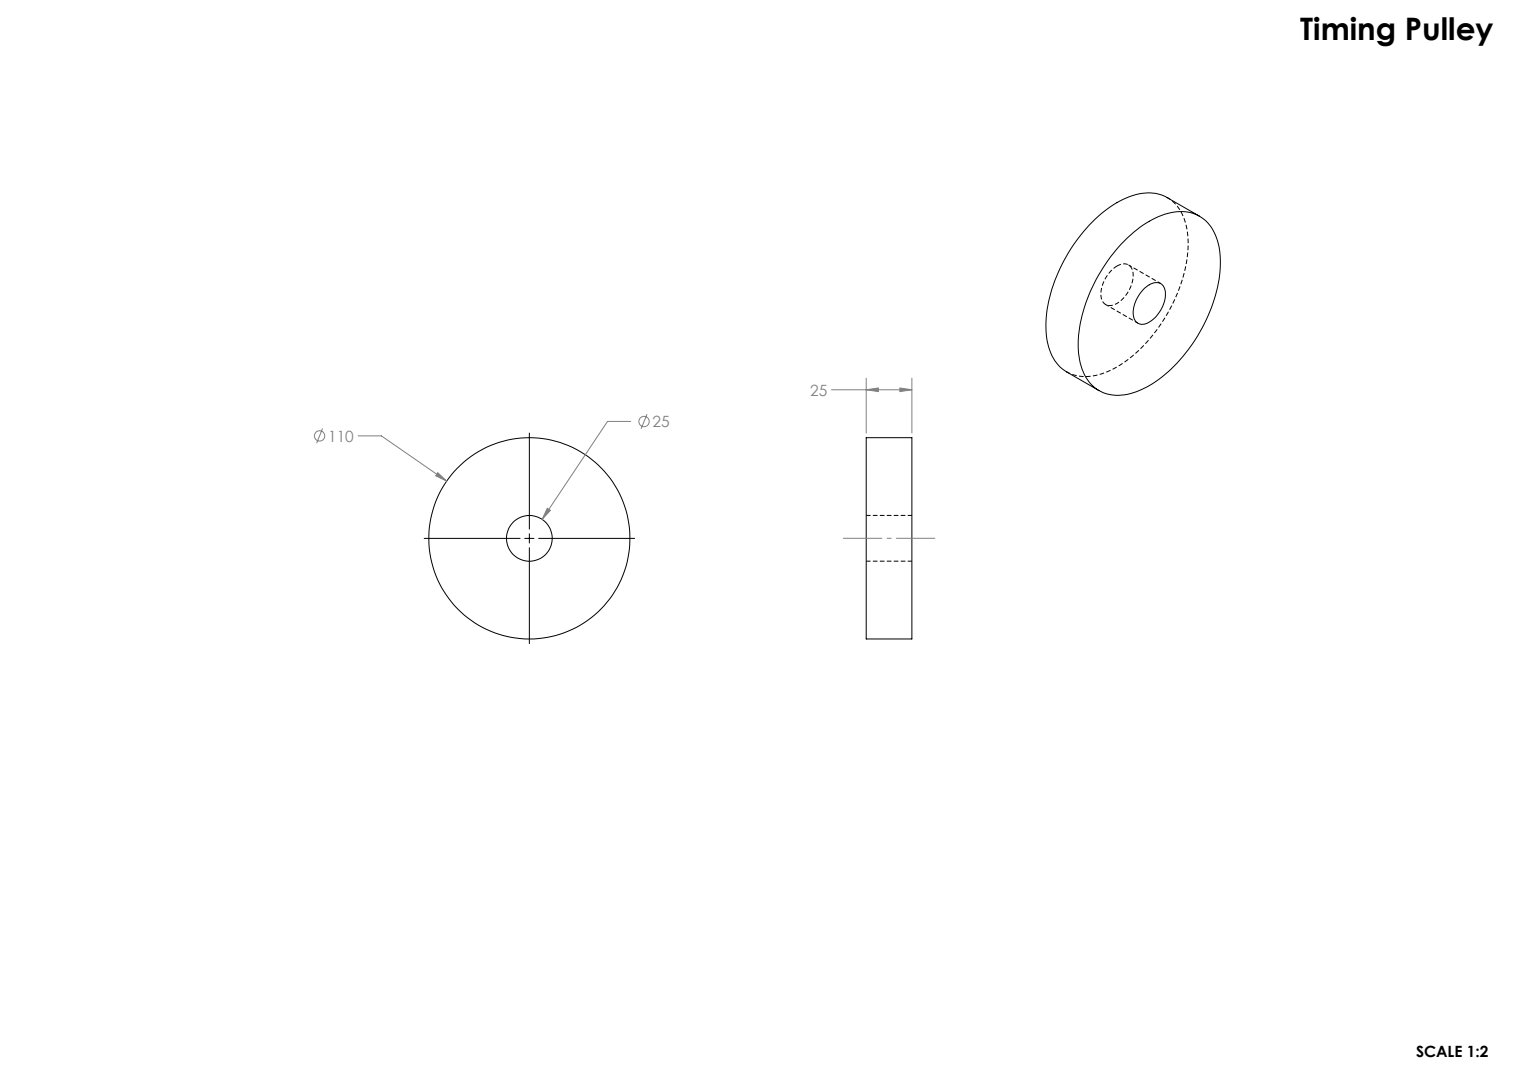
ISO-10303-21;
HEADER;
FILE_DESCRIPTION (('STEP AP214'),
    '1' );
FILE_NAME ('Timing Pulley.step',
    '2026-10-28T15:55:38',
    ( '' ),
    ( '' ),
    'SwSTEP 2.0',
    'SolidWorks 2025',
    '' );
FILE_SCHEMA (( 'AUTOMOTIVE_DESIGN' ));
ENDSEC;

DATA;
#97=ADVANCED_FACE ( 'NONE', ( #330, #202 ), #6713, .F. ) ;
#161=CARTESIAN_POINT ( 'NONE',  ( 5.551115123125782702E-14, 12.49999999999999645, -1.387778780781445676E-14 ) ) ;
#202=FACE_OUTER_BOUND ( 'NONE', #7839, .T. ) ;
#330=FACE_BOUND ( 'NONE', #1932, .T. ) ;
#354=VERTEX_POINT ( 'NONE', #1827 ) ;
#402=VERTEX_POINT ( 'NONE', #4592 ) ;
#516=AXIS2_PLACEMENT_3D ( 'NONE', #7483, #1692, #2897 ) ;
#543=CARTESIAN_POINT ( 'NONE',  ( 5.551115123125782702E-14, 12.49999999999999645, -1.387778780781445676E-14 ) ) ;
#563=AXIS2_PLACEMENT_3D ( 'NONE', #1559, #5435, #1598 ) ;
#639=AXIS2_PLACEMENT_3D ( 'NONE', #5635, #1167, #8220 ) ;
#714=DIRECTION ( 'NONE',  ( -1.752490724247359037E-17, 1.000000000000000000, 3.853078496550133260E-17 ) ) ;
#722=CARTESIAN_POINT ( 'NONE',  ( 5.551115123125782702E-14, 12.50000000000001066, -1.387778780781445676E-14 ) ) ;
#835=CARTESIAN_POINT ( 'NONE',  ( -1.173433385984103696E-13, -12.50000000000001066, -12.49999999999998757 ) ) ;
#854=VECTOR ( 'NONE', #4682, 1000.000000000000000 ) ;
#961=DIRECTION ( 'NONE',  ( 6.106226635438364917E-16, 3.154042683594196846E-17, 1.000000000000000000 ) ) ;
#969=PRODUCT_DEFINITION ( 'UNKNOWN', '', #7047, #8011 ) ;
#1020=ORIENTED_EDGE ( 'NONE', *, *, #2382, .F. ) ;
#1091=PRODUCT ( 'Timing Pulley', 'Timing Pulley', '', ( #7475 ) ) ;
#1167=DIRECTION ( 'NONE',  ( -1.752490724247359037E-17, 1.000000000000000000, 3.853078496550133260E-17 ) ) ;
#1272=CARTESIAN_POINT ( 'NONE',  ( -1.033895191682177028E-13, -12.50000000000001066, 12.50000000000000533 ) ) ;
#1299=AXIS2_PLACEMENT_3D ( 'NONE', #5884, #1507, #5927 ) ;
#1302=FACE_OUTER_BOUND ( 'NONE', #2125, .T. ) ;
#1306=CARTESIAN_POINT ( 'NONE',  ( -1.380900529026473240E-13, 12.49999999999999822, -55.00000000000001421 ) ) ;
#1313=ORIENTED_EDGE ( 'NONE', *, *, #1691, .T. ) ;
#1380=( LENGTH_UNIT ( ) NAMED_UNIT ( * ) SI_UNIT ( .MILLI., .METRE. ) );
#1422=ORIENTED_EDGE ( 'NONE', *, *, #7530, .F. ) ;
#1442=DIRECTION ( 'NONE',  ( 6.106226635438361958E-16, 0.000000000000000000, 1.000000000000000000 ) ) ;
#1481=( GEOMETRIC_REPRESENTATION_CONTEXT ( 3 ) GLOBAL_UNCERTAINTY_ASSIGNED_CONTEXT ( ( #5648 ) ) GLOBAL_UNIT_ASSIGNED_CONTEXT ( ( #2505, #4543, #3802 ) ) REPRESENTATION_CONTEXT ( 'NONE', 'WORKASPACE' ) );
#1501=ORIENTED_EDGE ( 'NONE', *, *, #6382, .F. ) ;
#1507=DIRECTION ( 'NONE',  ( 0.000000000000000000, 0.000000000000000000, 1.000000000000000000 ) ) ;
#1530=AXIS2_PLACEMENT_3D ( 'NONE', #2669, #2062, #2013 ) ;
#1559=CARTESIAN_POINT ( 'NONE',  ( -1.110223024625156540E-13, -12.49999999999999645, 1.387778780781445676E-14 ) ) ;
#1592=FACE_OUTER_BOUND ( 'NONE', #3238, .T. ) ;
#1598=DIRECTION ( 'NONE',  ( -6.106226635438364917E-16, -3.853078496550153598E-17, -1.000000000000000000 ) ) ;
#1650=DIRECTION ( 'NONE',  ( 6.106226635438361958E-16, 0.000000000000000000, 1.000000000000000000 ) ) ;
#1691=EDGE_CURVE ( 'NONE', #5627, #402, #6915, .T. ) ;
#1692=DIRECTION ( 'NONE',  ( -1.752490724247359037E-17, 1.000000000000000000, 3.853078496550133260E-17 ) ) ;
#1704=AXIS2_PLACEMENT_3D ( 'NONE', #2605, #5723, #8304 ) ;
#1705=DIRECTION ( 'NONE',  ( -1.752490724247359037E-17, 1.000000000000000000, 3.853078496550133260E-17 ) ) ;
#1733=VECTOR ( 'NONE', #5059, 1000.000000000000000 ) ;
#1752=ADVANCED_FACE ( 'NONE', ( #7099 ), #3846, .F. ) ;
#1780=EDGE_CURVE ( 'NONE', #5976, #2287, #7789, .T. ) ;
#1803=EDGE_CURVE ( 'NONE', #2287, #6267, #4623, .T. ) ;
#1827=CARTESIAN_POINT ( 'NONE',  ( -7.743805596760466869E-14, -12.49999999999999467, 54.99999999999997868 ) ) ;
#1884=CIRCLE ( 'NONE', #2423, 12.49999999999999289 ) ;
#1917=CARTESIAN_POINT ( 'NONE',  ( -7.743805596760466869E-14, -12.50000000000000888, 54.99999999999997868 ) ) ;
#1932=EDGE_LOOP ( 'NONE', ( #5556, #4034 ) ) ;
#1968=EDGE_CURVE ( 'NONE', #6651, #8339, #1884, .T. ) ;
#2013=DIRECTION ( 'NONE',  ( 6.106226635438364917E-16, 3.154042683594196846E-17, 1.000000000000000000 ) ) ;
#2062=DIRECTION ( 'NONE',  ( -1.752490724247359037E-17, 1.000000000000000000, 3.853078496550133260E-17 ) ) ;
#2125=EDGE_LOOP ( 'NONE', ( #7392, #3168, #5494, #5366 ) ) ;
#2287=VERTEX_POINT ( 'NONE', #1306 ) ;
#2300=CARTESIAN_POINT ( 'NONE',  ( 8.909539772616881237E-14, 12.49999999999999822, 54.99999999999995026 ) ) ;
#2382=EDGE_CURVE ( 'NONE', #402, #5627, #4177, .T. ) ;
#2398=ADVANCED_FACE ( 'NONE', ( #5522, #3511 ), #8130, .T. ) ;
#2423=AXIS2_PLACEMENT_3D ( 'NONE', #5830, #5321, #1442 ) ;
#2481=APPLICATION_CONTEXT ( 'automotive_design' ) ;
#2505=( LENGTH_UNIT ( ) NAMED_UNIT ( * ) SI_UNIT ( .MILLI., .METRE. ) );
#2512=CARTESIAN_POINT ( 'NONE',  ( -1.110223024625156540E-13, -12.50000000000001066, 1.387778780781445676E-14 ) ) ;
#2605=CARTESIAN_POINT ( 'NONE',  ( -1.110223024625156540E-13, -12.50000000000001066, 1.387778780781445676E-14 ) ) ;
#2607=AXIS2_PLACEMENT_3D ( 'NONE', #2512, #5752, #7022 ) ;
#2669=CARTESIAN_POINT ( 'NONE',  ( 5.551115123125782702E-14, 12.49999999999999645, -1.387778780781445676E-14 ) ) ;
#2741=DIRECTION ( 'NONE',  ( 1.752490724247363967E-17, -1.000000000000000000, 3.853078496550152365E-17 ) ) ;
#2796=AXIS2_PLACEMENT_3D ( 'NONE', #4981, #714, #5818 ) ;
#2897=DIRECTION ( 'NONE',  ( 6.106226635438364917E-16, 3.154042683594196846E-17, 1.000000000000000000 ) ) ;
#2966=CARTESIAN_POINT ( 'NONE',  ( -1.110223024625156540E-13, -12.50000000000001066, 1.387778780781445676E-14 ) ) ;
#3035=ADVANCED_FACE ( 'NONE', ( #1302 ), #6484, .T. ) ;
#3112=DIRECTION ( 'NONE',  ( -1.752490724247359037E-17, 1.000000000000000000, 3.853078496550133260E-17 ) ) ;
#3121=DIRECTION ( 'NONE',  ( -1.752490724247359037E-17, 1.000000000000000000, 3.853078496550133260E-17 ) ) ;
#3140=CYLINDRICAL_SURFACE ( 'NONE', #1704, 12.49999999999999289 ) ;
#3168=ORIENTED_EDGE ( 'NONE', *, *, #1780, .T. ) ;
#3185=UNCERTAINTY_MEASURE_WITH_UNIT (LENGTH_MEASURE( 1.000000000000000082E-05 ), #1380, 'distance_accuracy_value', 'NONE');
#3238=EDGE_LOOP ( 'NONE', ( #3403, #5267, #6886, #7093 ) ) ;
#3273=ORIENTED_EDGE ( 'NONE', *, *, #2382, .T. ) ;
#3372=ADVANCED_FACE ( 'NONE', ( #6988 ), #3140, .F. ) ;
#3403=ORIENTED_EDGE ( 'NONE', *, *, #1780, .F. ) ;
#3486=MECHANICAL_DESIGN_GEOMETRIC_PRESENTATION_REPRESENTATION('',(#7953),#1481);
#3511=FACE_OUTER_BOUND ( 'NONE', #5551, .T. ) ;
#3621=EDGE_LOOP ( 'NONE', ( #3273, #1313 ) ) ;
#3632=( NAMED_UNIT ( * ) PLANE_ANGLE_UNIT ( ) SI_UNIT ( $, .RADIAN. ) );
#3648=AXIS2_PLACEMENT_3D ( 'NONE', #3919, #6487, #4834 ) ;
#3708=PRODUCT_DEFINITION_SHAPE ( 'NONE', 'NONE',  #969 ) ;
#3729=CIRCLE ( 'NONE', #5885, 12.49999999999999289 ) ;
#3802=( NAMED_UNIT ( * ) SI_UNIT ( $, .STERADIAN. ) SOLID_ANGLE_UNIT ( ) );
#3846=CYLINDRICAL_SURFACE ( 'NONE', #2607, 12.49999999999999289 ) ;
#3890=CARTESIAN_POINT ( 'NONE',  ( -1.380900529026471473E-13, -12.49999999999999467, -54.99999999999998579 ) ) ;
#3905=CARTESIAN_POINT ( 'NONE',  ( -1.173433385984108997E-13, 12.50000000000001066, -12.50000000000001421 ) ) ;
#3919=CARTESIAN_POINT ( 'NONE',  ( -1.110223024625156540E-13, -12.50000000000001066, 1.387778780781445676E-14 ) ) ;
#3930=EDGE_CURVE ( 'NONE', #8339, #6651, #3729, .T. ) ;
#3965=SHAPE_REPRESENTATION ( 'Timing Pulley', ( #1299 ), #6550 ) ;
#3985=DIRECTION ( 'NONE',  ( -1.752490724247359037E-17, 1.000000000000000000, 3.853078496550133260E-17 ) ) ;
#4034=ORIENTED_EDGE ( 'NONE', *, *, #3930, .F. ) ;
#4091=EDGE_CURVE ( 'NONE', #354, #5976, #7375, .T. ) ;
#4132=CIRCLE ( 'NONE', #516, 54.99999999999996447 ) ;
#4177=CIRCLE ( 'NONE', #3648, 12.49999999999999289 ) ;
#4463=DIRECTION ( 'NONE',  ( 6.106226635438361958E-16, 0.000000000000000000, 1.000000000000000000 ) ) ;
#4480=CLOSED_SHELL ( 'NONE', ( #3035, #1752, #2398, #3372, #97, #5773 ) ) ;
#4541=LINE ( 'NONE', #1917, #1733 ) ;
#4543=( NAMED_UNIT ( * ) PLANE_ANGLE_UNIT ( ) SI_UNIT ( $, .RADIAN. ) );
#4581=ORIENTED_EDGE ( 'NONE', *, *, #4956, .F. ) ;
#4592=CARTESIAN_POINT ( 'NONE',  ( -1.033895191682177028E-13, -12.50000000000001066, 12.50000000000000533 ) ) ;
#4623=CIRCLE ( 'NONE', #1530, 54.99999999999996447 ) ;
#4666=ORIENTED_EDGE ( 'NONE', *, *, #6382, .T. ) ;
#4682=DIRECTION ( 'NONE',  ( -1.752490724247359037E-17, 1.000000000000000000, 3.853078496550133260E-17 ) ) ;
#4708=VECTOR ( 'NONE', #1705, 1000.000000000000000 ) ;
#4721=CARTESIAN_POINT ( 'NONE',  ( -1.110223024625156540E-13, -12.50000000000001066, 1.387778780781445676E-14 ) ) ;
#4764=DIRECTION ( 'NONE',  ( -6.106226635438364917E-16, -3.853078496550153598E-17, -1.000000000000000000 ) ) ;
#4834=DIRECTION ( 'NONE',  ( 6.106226635438361958E-16, 0.000000000000000000, 1.000000000000000000 ) ) ;
#4863=( NAMED_UNIT ( * ) SI_UNIT ( $, .STERADIAN. ) SOLID_ANGLE_UNIT ( ) );
#4956=EDGE_CURVE ( 'NONE', #5976, #354, #4132, .T. ) ;
#4966=AXIS2_PLACEMENT_3D ( 'NONE', #2966, #8003, #961 ) ;
#4981=CARTESIAN_POINT ( 'NONE',  ( -1.110223024625156540E-13, -12.50000000000001066, 1.387778780781445676E-14 ) ) ;
#5022=AXIS2_PLACEMENT_3D ( 'NONE', #4721, #6670, #1650 ) ;
#5059=DIRECTION ( 'NONE',  ( -1.752490724247359037E-17, 1.000000000000000000, 3.853078496550133260E-17 ) ) ;
#5061=ORIENTED_EDGE ( 'NONE', *, *, #7530, .T. ) ;
#5100=EDGE_CURVE ( 'NONE', #354, #6267, #4541, .T. ) ;
#5267=ORIENTED_EDGE ( 'NONE', *, *, #4956, .T. ) ;
#5321=DIRECTION ( 'NONE',  ( -1.752490724247359037E-17, 1.000000000000000000, 3.853078496550133260E-17 ) ) ;
#5366=ORIENTED_EDGE ( 'NONE', *, *, #5100, .F. ) ;
#5435=DIRECTION ( 'NONE',  ( 1.752490724247363967E-17, -1.000000000000000000, 3.853078496550152365E-17 ) ) ;
#5494=ORIENTED_EDGE ( 'NONE', *, *, #5515, .F. ) ;
#5505=LINE ( 'NONE', #6079, #4708 ) ;
#5515=EDGE_CURVE ( 'NONE', #6267, #2287, #8218, .T. ) ;
#5522=FACE_BOUND ( 'NONE', #3621, .T. ) ;
#5551=EDGE_LOOP ( 'NONE', ( #6960, #4581 ) ) ;
#5554=CYLINDRICAL_SURFACE ( 'NONE', #4966, 54.99999999999996447 ) ;
#5556=ORIENTED_EDGE ( 'NONE', *, *, #1968, .F. ) ;
#5627=VERTEX_POINT ( 'NONE', #835 ) ;
#5635=CARTESIAN_POINT ( 'NONE',  ( -1.110223024625156540E-13, -12.49999999999999645, 1.387778780781445676E-14 ) ) ;
#5648=UNCERTAINTY_MEASURE_WITH_UNIT (LENGTH_MEASURE( 1.000000000000000082E-05 ), #2505, 'distance_accuracy_value', 'NONE');
#5702=LINE ( 'NONE', #1272, #6053 ) ;
#5723=DIRECTION ( 'NONE',  ( -1.752490724247359037E-17, 1.000000000000000000, 3.853078496550133260E-17 ) ) ;
#5752=DIRECTION ( 'NONE',  ( -1.752490724247359037E-17, 1.000000000000000000, 3.853078496550133260E-17 ) ) ;
#5773=ADVANCED_FACE ( 'NONE', ( #1592 ), #5554, .T. ) ;
#5818=DIRECTION ( 'NONE',  ( 6.106226635438364917E-16, 3.154042683594196846E-17, 1.000000000000000000 ) ) ;
#5830=CARTESIAN_POINT ( 'NONE',  ( 5.551115123125782702E-14, 12.50000000000001066, -1.387778780781445676E-14 ) ) ;
#5860=APPLICATION_CONTEXT ( 'automotive_design' ) ;
#5884=CARTESIAN_POINT ( 'NONE',  ( 0.000000000000000000, 0.000000000000000000, 0.000000000000000000 ) ) ;
#5885=AXIS2_PLACEMENT_3D ( 'NONE', #722, #3985, #4463 ) ;
#5907=AXIS2_PLACEMENT_3D ( 'NONE', #543, #3112, #6359 ) ;
#5927=DIRECTION ( 'NONE',  ( 1.000000000000000000, 0.000000000000000000, 0.000000000000000000 ) ) ;
#5976=VERTEX_POINT ( 'NONE', #3890 ) ;
#6053=VECTOR ( 'NONE', #3121, 1000.000000000000000 ) ;
#6079=CARTESIAN_POINT ( 'NONE',  ( -1.171242772578794285E-13, -12.50000000000001066, -12.49999999999997868 ) ) ;
#6087=ORIENTED_EDGE ( 'NONE', *, *, #1691, .F. ) ;
#6158=ORIENTED_EDGE ( 'NONE', *, *, #3930, .T. ) ;
#6267=VERTEX_POINT ( 'NONE', #2300 ) ;
#6284=EDGE_LOOP ( 'NONE', ( #1422, #1020, #4666, #7192 ) ) ;
#6292=ORIENTED_EDGE ( 'NONE', *, *, #1803, .T. ) ;
#6359=DIRECTION ( 'NONE',  ( 6.106226635438364917E-16, 3.154042683594196846E-17, 1.000000000000000000 ) ) ;
#6382=EDGE_CURVE ( 'NONE', #402, #6651, #5702, .T. ) ;
#6411=MANIFOLD_SOLID_BREP ( 'Revolve1', #4480 ) ;
#6484=CYLINDRICAL_SURFACE ( 'NONE', #2796, 54.99999999999996447 ) ;
#6487=DIRECTION ( 'NONE',  ( -1.752490724247359037E-17, 1.000000000000000000, 3.853078496550133260E-17 ) ) ;
#6550=( GEOMETRIC_REPRESENTATION_CONTEXT ( 3 ) GLOBAL_UNCERTAINTY_ASSIGNED_CONTEXT ( ( #3185 ) ) GLOBAL_UNIT_ASSIGNED_CONTEXT ( ( #1380, #3632, #4863 ) ) REPRESENTATION_CONTEXT ( 'NONE', 'WORKASPACE' ) );
#6651=VERTEX_POINT ( 'NONE', #7472 ) ;
#6670=DIRECTION ( 'NONE',  ( -1.752490724247359037E-17, 1.000000000000000000, 3.853078496550133260E-17 ) ) ;
#6713=PLANE ( 'NONE',  #7329 ) ;
#6886=ORIENTED_EDGE ( 'NONE', *, *, #5100, .T. ) ;
#6915=CIRCLE ( 'NONE', #5022, 12.49999999999999289 ) ;
#6960=ORIENTED_EDGE ( 'NONE', *, *, #4091, .F. ) ;
#6988=FACE_OUTER_BOUND ( 'NONE', #6284, .T. ) ;
#7022=DIRECTION ( 'NONE',  ( 6.106226635438361958E-16, 0.000000000000000000, 1.000000000000000000 ) ) ;
#7047=PRODUCT_DEFINITION_FORMATION_WITH_SPECIFIED_SOURCE ( 'ANY', '', #1091, .NOT_KNOWN. ) ;
#7093=ORIENTED_EDGE ( 'NONE', *, *, #1803, .F. ) ;
#7099=FACE_OUTER_BOUND ( 'NONE', #7404, .T. ) ;
#7192=ORIENTED_EDGE ( 'NONE', *, *, #1968, .T. ) ;
#7329=AXIS2_PLACEMENT_3D ( 'NONE', #161, #2741, #4764 ) ;
#7375=CIRCLE ( 'NONE', #639, 54.99999999999996447 ) ;
#7392=ORIENTED_EDGE ( 'NONE', *, *, #4091, .T. ) ;
#7404=EDGE_LOOP ( 'NONE', ( #6087, #5061, #6158, #1501 ) ) ;
#7431=ORIENTED_EDGE ( 'NONE', *, *, #5515, .T. ) ;
#7472=CARTESIAN_POINT ( 'NONE',  ( 6.314393452555577824E-14, 12.50000000000001066, 12.49999999999997868 ) ) ;
#7475=PRODUCT_CONTEXT ( 'NONE', #5860, 'mechanical' ) ;
#7483=CARTESIAN_POINT ( 'NONE',  ( -1.110223024625156540E-13, -12.49999999999999645, 1.387778780781445676E-14 ) ) ;
#7530=EDGE_CURVE ( 'NONE', #5627, #8339, #5505, .T. ) ;
#7639=ADVANCED_BREP_SHAPE_REPRESENTATION ( '', ( #6411, #1299 ), #6550 ) ;
#7789=LINE ( 'NONE', #7836, #854 ) ;
#7836=CARTESIAN_POINT ( 'NONE',  ( -1.378709915621162062E-13, -12.50000000000001243, -54.99999999999995026 ) ) ;
#7839=EDGE_LOOP ( 'NONE', ( #7431, #6292 ) ) ;
#7953=STYLED_ITEM('',(#8414),#6411);
#8003=DIRECTION ( 'NONE',  ( -1.752490724247359037E-17, 1.000000000000000000, 3.853078496550133260E-17 ) ) ;
#8011=PRODUCT_DEFINITION_CONTEXT ( 'detailed design', #2481, 'design' ) ;
#8118=SHAPE_REPRESENTATION_RELATIONSHIP ( 'NONE' , 'NONE' ,  #3965, #7639 ) ;
#8130=PLANE ( 'NONE',  #563 ) ;
#8218=CIRCLE ( 'NONE', #5907, 54.99999999999996447 ) ;
#8220=DIRECTION ( 'NONE',  ( 6.106226635438364917E-16, 3.154042683594196846E-17, 1.000000000000000000 ) ) ;
#8237=SHAPE_DEFINITION_REPRESENTATION ( #3708, #3965 ) ;
#8304=DIRECTION ( 'NONE',  ( 6.106226635438361958E-16, 0.000000000000000000, 1.000000000000000000 ) ) ;
#8339=VERTEX_POINT ( 'NONE', #3905 ) ;
#8408=COLOUR_RGB('Off White',0.89,0.88,0.83);
#8409=FILL_AREA_STYLE_COLOUR('',#8408);
#8410=FILL_AREA_STYLE('',(#8409));
#8411=SURFACE_STYLE_FILL_AREA(#8410);
#8412=SURFACE_SIDE_STYLE('',(#8411));
#8413=SURFACE_STYLE_USAGE(.BOTH.,#8412);
#8414=PRESENTATION_STYLE_ASSIGNMENT((#8413));
ENDSEC;
END-ISO-10303-21;
